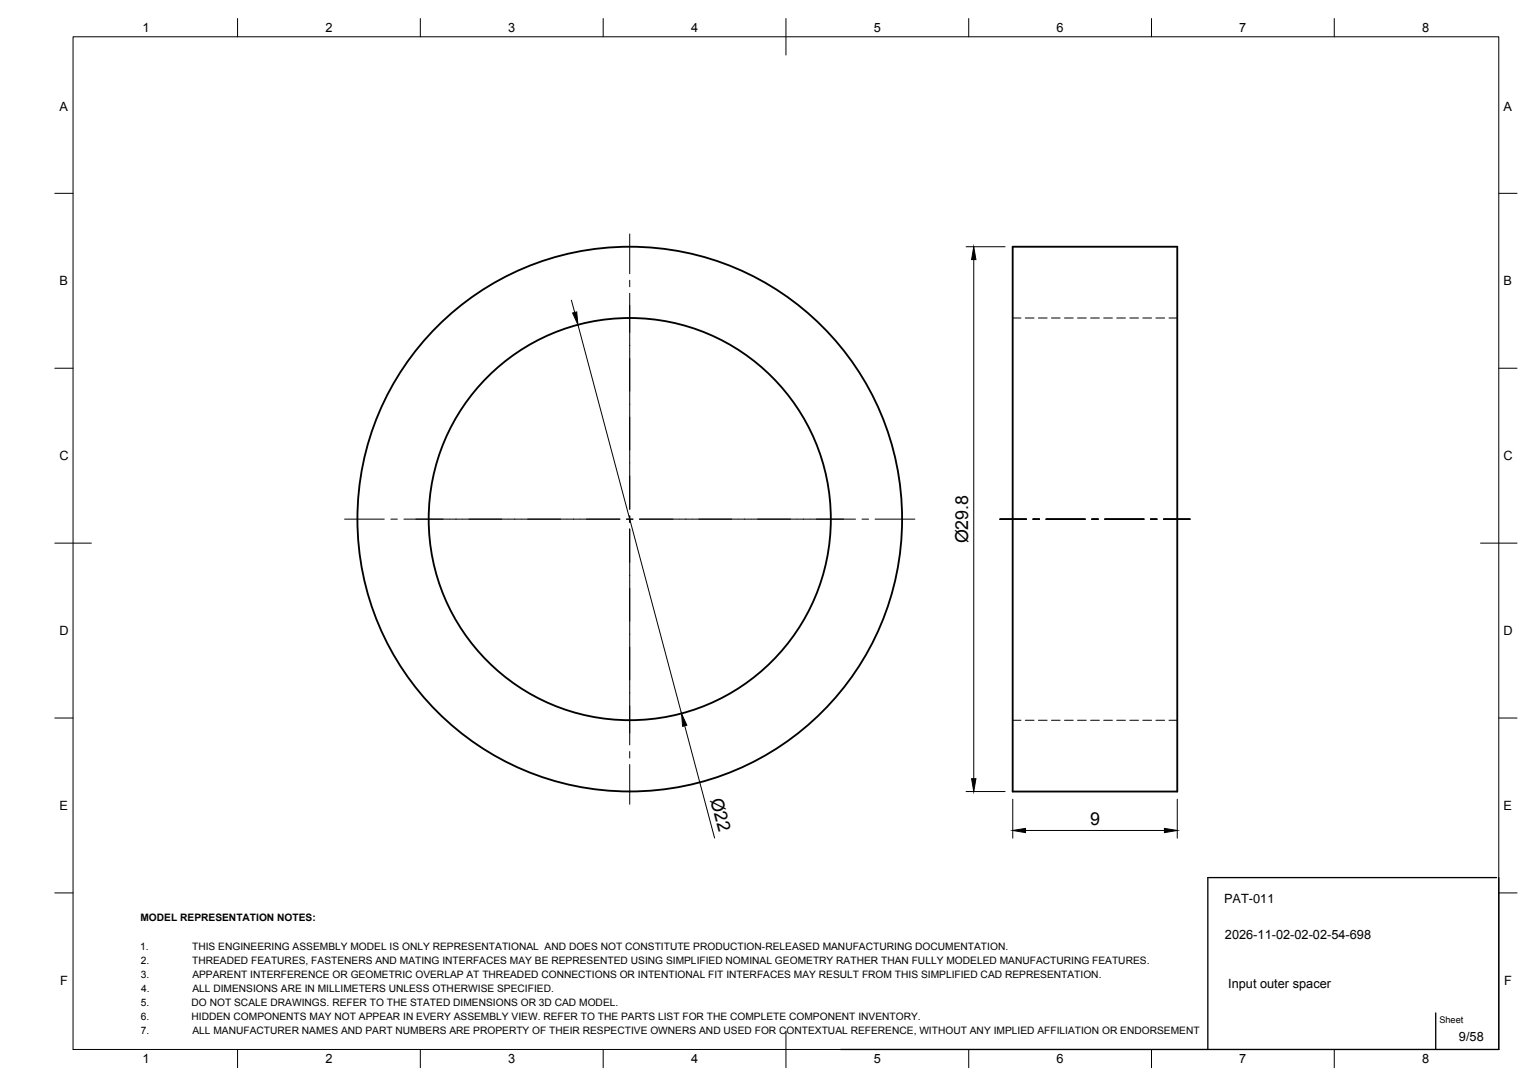
ISO-10303-21;
HEADER;
/* Generated by software containing ST-Developer
 * from STEP Tools, Inc. (www.steptools.com) 
 */

FILE_DESCRIPTION(
/* description */ ('Belt tension measurement rig'),
/* implementation_level */ '2;1');

FILE_NAME(
/* name */ 'Input outer spacer.step',
/* time_stamp */ '2026-10-28T03:24:44-07:00',
/* author */ (''),
/* organization */ (''),
/* preprocessor_version */ 'ST-DEVELOPER v20.2',
/* originating_system */ 'Autodesk Translation Framework v15.17.0.0',
/* authorisation */ '');

FILE_SCHEMA (('AUTOMOTIVE_DESIGN { 1 0 10303 214 3 1 1 }'));
ENDSEC;

DATA;
#10=MECHANICAL_DESIGN_GEOMETRIC_PRESENTATION_REPRESENTATION('',(#696),#23587);
#586=SHAPE_REPRESENTATION_RELATIONSHIP('SRR','None',#23831,#641);
#641=ADVANCED_BREP_SHAPE_REPRESENTATION('',(#766),#23529);
#696=STYLED_ITEM('',(#24204),#766);
#766=MANIFOLD_SOLID_BREP('Body1',#12201);
#861=FACE_BOUND('',#2156,.T.);
#862=FACE_BOUND('',#2158,.T.);
#1079=PLANE('',#13000);
#1080=PLANE('',#13001);
#1417=FACE_OUTER_BOUND('',#2153,.T.);
#1418=FACE_OUTER_BOUND('',#2154,.T.);
#1419=FACE_OUTER_BOUND('',#2155,.T.);
#1420=FACE_OUTER_BOUND('',#2157,.T.);
#2153=EDGE_LOOP('',(#8196,#8197,#8198,#8199));
#2154=EDGE_LOOP('',(#8200,#8201,#8202,#8203));
#2155=EDGE_LOOP('',(#8204));
#2156=EDGE_LOOP('',(#8205));
#2157=EDGE_LOOP('',(#8206));
#2158=EDGE_LOOP('',(#8207));
#3051=LINE('',#18841,#3802);
#3052=LINE('',#18847,#3803);
#3802=VECTOR('',#14840,1.1);
#3803=VECTOR('',#14847,1.49);
#4516=CIRCLE('',#12995,1.1);
#4517=CIRCLE('',#12996,1.1);
#4518=CIRCLE('',#12998,1.49);
#4519=CIRCLE('',#12999,1.49);
#5324=VERTEX_POINT('',#18838);
#5325=VERTEX_POINT('',#18840);
#5326=VERTEX_POINT('',#18844);
#5327=VERTEX_POINT('',#18846);
#6457=EDGE_CURVE('',#5324,#5324,#4516,.T.);
#6458=EDGE_CURVE('',#5324,#5325,#3051,.T.);
#6459=EDGE_CURVE('',#5325,#5325,#4517,.T.);
#6460=EDGE_CURVE('',#5326,#5326,#4518,.T.);
#6461=EDGE_CURVE('',#5326,#5327,#3052,.T.);
#6462=EDGE_CURVE('',#5327,#5327,#4519,.T.);
#8196=ORIENTED_EDGE('',*,*,#6457,.F.);
#8197=ORIENTED_EDGE('',*,*,#6458,.T.);
#8198=ORIENTED_EDGE('',*,*,#6459,.T.);
#8199=ORIENTED_EDGE('',*,*,#6458,.F.);
#8200=ORIENTED_EDGE('',*,*,#6460,.F.);
#8201=ORIENTED_EDGE('',*,*,#6461,.T.);
#8202=ORIENTED_EDGE('',*,*,#6462,.T.);
#8203=ORIENTED_EDGE('',*,*,#6461,.F.);
#8204=ORIENTED_EDGE('',*,*,#6460,.T.);
#8205=ORIENTED_EDGE('',*,*,#6457,.T.);
#8206=ORIENTED_EDGE('',*,*,#6462,.F.);
#8207=ORIENTED_EDGE('',*,*,#6459,.F.);
#11181=CYLINDRICAL_SURFACE('',#12994,1.1);
#11182=CYLINDRICAL_SURFACE('',#12997,1.49);
#11558=ADVANCED_FACE('',(#1417),#11181,.F.);
#11559=ADVANCED_FACE('',(#1418),#11182,.T.);
#11560=ADVANCED_FACE('',(#1419,#861),#1079,.T.);
#11561=ADVANCED_FACE('',(#1420,#862),#1080,.F.);
#12201=CLOSED_SHELL('',(#11558,#11559,#11560,#11561));
#12993=AXIS2_PLACEMENT_3D('',#18836,#14834,#14835);
#12994=AXIS2_PLACEMENT_3D('',#18837,#14836,#14837);
#12995=AXIS2_PLACEMENT_3D('',#18839,#14838,#14839);
#12996=AXIS2_PLACEMENT_3D('',#18842,#14841,#14842);
#12997=AXIS2_PLACEMENT_3D('',#18843,#14843,#14844);
#12998=AXIS2_PLACEMENT_3D('',#18845,#14845,#14846);
#12999=AXIS2_PLACEMENT_3D('',#18848,#14848,#14849);
#13000=AXIS2_PLACEMENT_3D('',#18849,#14850,#14851);
#13001=AXIS2_PLACEMENT_3D('',#18850,#14852,#14853);
#14834=DIRECTION('axis',(0.,0.,1.));
#14835=DIRECTION('refdir',(1.,0.,0.));
#14836=DIRECTION('center_axis',(0.,1.,0.));
#14837=DIRECTION('ref_axis',(1.,0.,0.));
#14838=DIRECTION('center_axis',(0.,-1.,0.));
#14839=DIRECTION('ref_axis',(1.,0.,0.));
#14840=DIRECTION('',(0.,-1.,0.));
#14841=DIRECTION('center_axis',(0.,-1.,0.));
#14842=DIRECTION('ref_axis',(1.,0.,0.));
#14843=DIRECTION('center_axis',(0.,1.,0.));
#14844=DIRECTION('ref_axis',(1.,0.,0.));
#14845=DIRECTION('center_axis',(0.,1.,0.));
#14846=DIRECTION('ref_axis',(1.,0.,0.));
#14847=DIRECTION('',(0.,-1.,0.));
#14848=DIRECTION('center_axis',(0.,1.,0.));
#14849=DIRECTION('ref_axis',(1.,0.,0.));
#14850=DIRECTION('center_axis',(0.,1.,0.));
#14851=DIRECTION('ref_axis',(1.,0.,0.));
#14852=DIRECTION('center_axis',(0.,1.,0.));
#14853=DIRECTION('ref_axis',(1.,0.,0.));
#18836=CARTESIAN_POINT('',(0.,0.,0.));
#18837=CARTESIAN_POINT('Origin',(0.,-0.45,7.));
#18838=CARTESIAN_POINT('',(-1.1,0.45,7.));
#18839=CARTESIAN_POINT('Origin',(0.,0.45,7.));
#18840=CARTESIAN_POINT('',(-1.1,-0.45,7.));
#18841=CARTESIAN_POINT('',(-1.1,-0.45,7.));
#18842=CARTESIAN_POINT('Origin',(0.,-0.45,7.));
#18843=CARTESIAN_POINT('Origin',(0.,-0.45,7.));
#18844=CARTESIAN_POINT('',(-1.49,0.45,7.));
#18845=CARTESIAN_POINT('Origin',(0.,0.45,7.));
#18846=CARTESIAN_POINT('',(-1.49,-0.45,7.));
#18847=CARTESIAN_POINT('',(-1.49,-0.45,7.));
#18848=CARTESIAN_POINT('Origin',(0.,-0.45,7.));
#18849=CARTESIAN_POINT('Origin',(0.,0.45,7.));
#18850=CARTESIAN_POINT('Origin',(0.,-0.45,7.));
#23464=UNCERTAINTY_MEASURE_WITH_UNIT(LENGTH_MEASURE(0.001),#23588,
'DISTANCE_ACCURACY_VALUE',
'Maximum model space distance between geometric entities at asserted c
onnectivities');
#23522=UNCERTAINTY_MEASURE_WITH_UNIT(LENGTH_MEASURE(0.001),#23588,
'DISTANCE_ACCURACY_VALUE',
'Maximum model space distance between geometric entities at asserted c
onnectivities');
#23529=(
GEOMETRIC_REPRESENTATION_CONTEXT(3)
GLOBAL_UNCERTAINTY_ASSIGNED_CONTEXT((#23464))
GLOBAL_UNIT_ASSIGNED_CONTEXT((#23588,#23590,#23591))
REPRESENTATION_CONTEXT('','3D')
);
#23587=(
GEOMETRIC_REPRESENTATION_CONTEXT(3)
GLOBAL_UNCERTAINTY_ASSIGNED_CONTEXT((#23522))
GLOBAL_UNIT_ASSIGNED_CONTEXT((#23588,#23590,#23591))
REPRESENTATION_CONTEXT('','3D')
);
#23588=(
LENGTH_UNIT()
NAMED_UNIT(*)
SI_UNIT(.CENTI.,.METRE.)
);
#23590=(
NAMED_UNIT(*)
PLANE_ANGLE_UNIT()
SI_UNIT($,.RADIAN.)
);
#23591=(
NAMED_UNIT(*)
SI_UNIT($,.STERADIAN.)
SOLID_ANGLE_UNIT()
);
#23598=SHAPE_DEFINITION_REPRESENTATION(#23662,#23831);
#23662=PRODUCT_DEFINITION_SHAPE('',$,#23896);
#23831=SHAPE_REPRESENTATION('',(#12993),#23529);
#23889=PRODUCT_DEFINITION_CONTEXT('part definition',#24083,'design');
#23896=PRODUCT_DEFINITION('Input outer spacer','Input outer spacer',#23960,
#23889);
#23960=PRODUCT_DEFINITION_FORMATION('',$,#24091);
#24083=APPLICATION_CONTEXT(
'Core Data for Automotive Mechanical Design Process');
#24084=PRODUCT_CONTEXT('part definition',#24083,'mechanical');
#24091=PRODUCT('Input outer spacer','Input outer spacer',
'Input outer spacer',(#24084));
#24198=COLOUR_RGB('Sky Blue',0.24,0.69,0.87);
#24199=FILL_AREA_STYLE_COLOUR('',#24198);
#24200=FILL_AREA_STYLE('',(#24199));
#24201=SURFACE_STYLE_FILL_AREA(#24200);
#24202=SURFACE_SIDE_STYLE('',(#24201));
#24203=SURFACE_STYLE_USAGE(.BOTH.,#24202);
#24204=PRESENTATION_STYLE_ASSIGNMENT((#24203));
ENDSEC;
END-ISO-10303-21;
